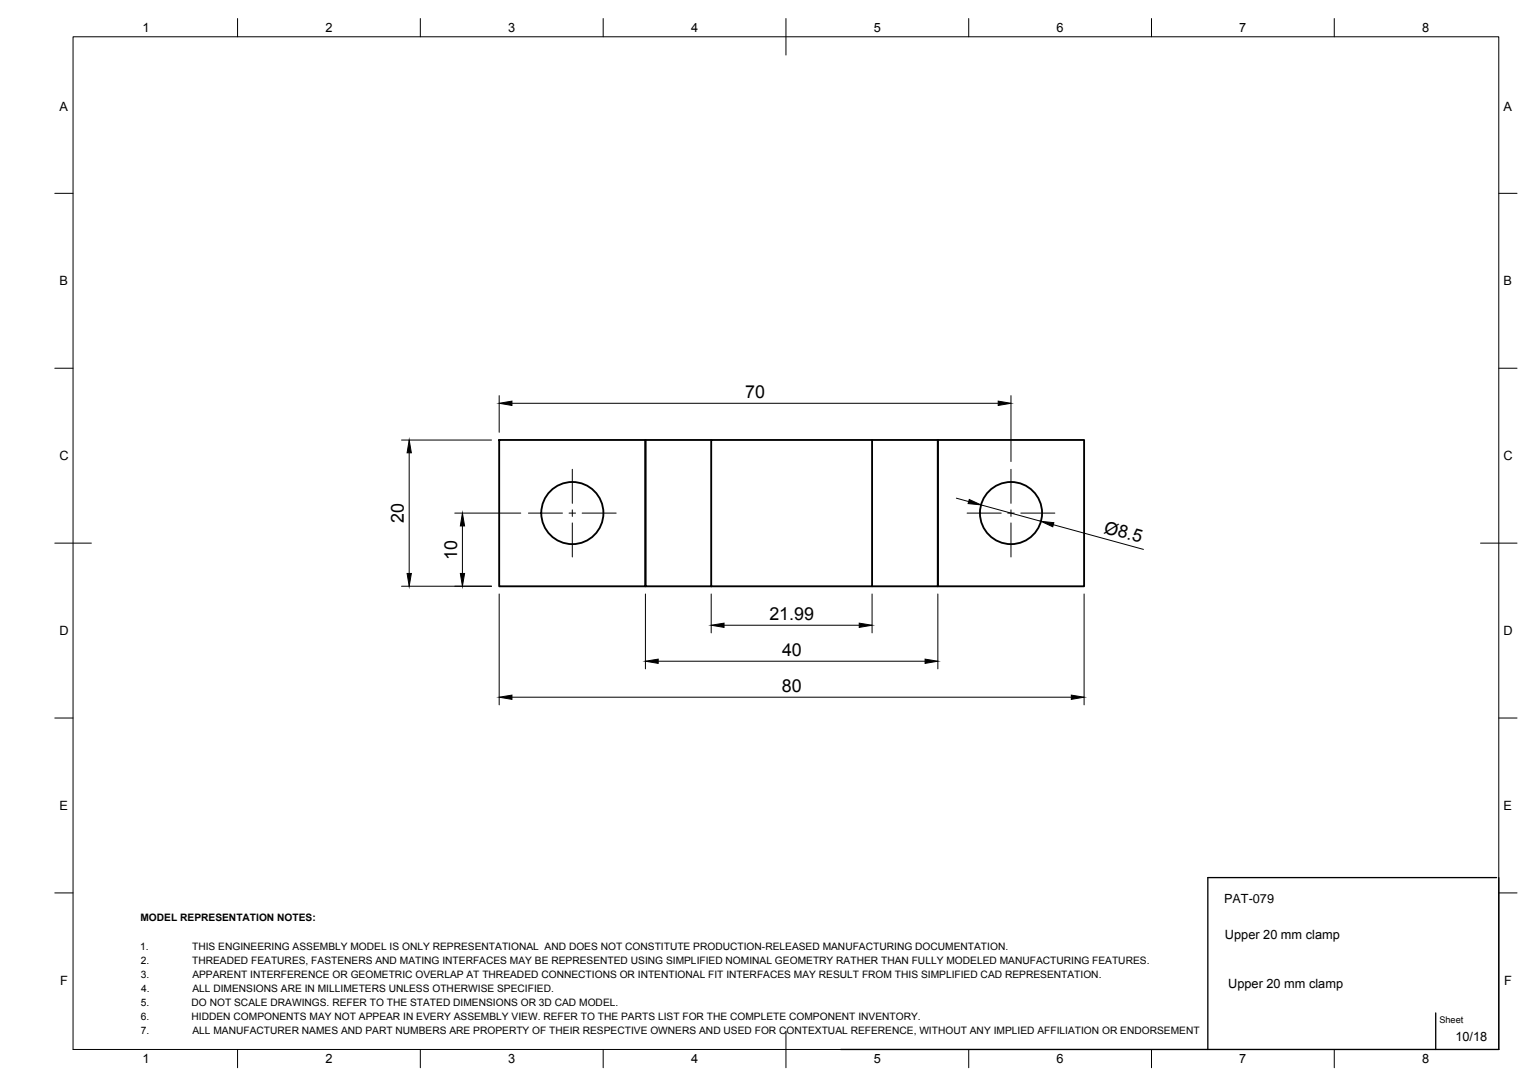
ISO-10303-21;
HEADER;
/* Generated by software containing ST-Developer
 * from STEP Tools, Inc. (www.steptools.com) 
 */

FILE_DESCRIPTION(
/* description */ ('Pipe clamp stand with threaded column'),
/* implementation_level */ '2;1');

FILE_NAME(
/* name */ 'Upper 20 mm clamp.step',
/* time_stamp */ '2026-10-27T10:55:48-07:00',
/* author */ (''),
/* organization */ (''),
/* preprocessor_version */ 'ST-DEVELOPER v20.2',
/* originating_system */ 'Autodesk Translation Framework v15.17.0.0',
/* authorisation */ '');

FILE_SCHEMA (('AUTOMOTIVE_DESIGN { 1 0 10303 214 3 1 1 }'));
ENDSEC;

DATA;
#10=MECHANICAL_DESIGN_GEOMETRIC_PRESENTATION_REPRESENTATION('',(#748,#749,#750),#34433);
#702=SHAPE_REPRESENTATION_RELATIONSHIP('SRR','None',#34544,#724);
#724=ADVANCED_BREP_SHAPE_REPRESENTATION('',(#778,#779,#780),#34412);
#748=STYLED_ITEM('',(#34729),#778);
#749=STYLED_ITEM('',(#34729),#779);
#750=STYLED_ITEM('',(#34729),#780);
#778=MANIFOLD_SOLID_BREP('Body1',#8775);
#779=MANIFOLD_SOLID_BREP('Body2',#8776);
#780=MANIFOLD_SOLID_BREP('Body3',#8777);
#828=FACE_BOUND('',#1821,.T.);
#829=FACE_BOUND('',#1824,.T.);
#830=FACE_BOUND('',#1830,.T.);
#831=FACE_BOUND('',#1833,.T.);
#895=PLANE('',#9352);
#896=PLANE('',#9354);
#897=PLANE('',#9355);
#898=PLANE('',#9358);
#899=PLANE('',#9362);
#900=PLANE('',#9363);
#901=PLANE('',#9364);
#902=PLANE('',#9365);
#903=PLANE('',#9366);
#904=PLANE('',#9367);
#905=PLANE('',#9371);
#906=PLANE('',#9372);
#907=PLANE('',#9373);
#908=PLANE('',#9374);
#909=PLANE('',#9375);
#910=PLANE('',#9376);
#1296=FACE_OUTER_BOUND('',#1812,.T.);
#1297=FACE_OUTER_BOUND('',#1813,.T.);
#1298=FACE_OUTER_BOUND('',#1814,.T.);
#1299=FACE_OUTER_BOUND('',#1815,.T.);
#1300=FACE_OUTER_BOUND('',#1816,.T.);
#1301=FACE_OUTER_BOUND('',#1817,.T.);
#1302=FACE_OUTER_BOUND('',#1818,.T.);
#1303=FACE_OUTER_BOUND('',#1819,.T.);
#1304=FACE_OUTER_BOUND('',#1820,.T.);
#1305=FACE_OUTER_BOUND('',#1822,.T.);
#1306=FACE_OUTER_BOUND('',#1823,.T.);
#1307=FACE_OUTER_BOUND('',#1825,.T.);
#1308=FACE_OUTER_BOUND('',#1826,.T.);
#1309=FACE_OUTER_BOUND('',#1827,.T.);
#1310=FACE_OUTER_BOUND('',#1828,.T.);
#1311=FACE_OUTER_BOUND('',#1829,.T.);
#1312=FACE_OUTER_BOUND('',#1831,.T.);
#1313=FACE_OUTER_BOUND('',#1832,.T.);
#1314=FACE_OUTER_BOUND('',#1834,.T.);
#1315=FACE_OUTER_BOUND('',#1835,.T.);
#1812=EDGE_LOOP('',(#6923,#6924,#6925,#6926));
#1813=EDGE_LOOP('',(#6927,#6928,#6929,#6930));
#1814=EDGE_LOOP('',(#6931,#6932,#6933,#6934));
#1815=EDGE_LOOP('',(#6935,#6936,#6937,#6938));
#1816=EDGE_LOOP('',(#6939,#6940,#6941,#6942));
#1817=EDGE_LOOP('',(#6943,#6944,#6945,#6946));
#1818=EDGE_LOOP('',(#6947,#6948,#6949,#6950));
#1819=EDGE_LOOP('',(#6951,#6952,#6953,#6954));
#1820=EDGE_LOOP('',(#6955,#6956,#6957,#6958));
#1821=EDGE_LOOP('',(#6959));
#1822=EDGE_LOOP('',(#6960,#6961,#6962,#6963));
#1823=EDGE_LOOP('',(#6964,#6965,#6966,#6967));
#1824=EDGE_LOOP('',(#6968));
#1825=EDGE_LOOP('',(#6969,#6970,#6971,#6972));
#1826=EDGE_LOOP('',(#6973,#6974,#6975,#6976));
#1827=EDGE_LOOP('',(#6977,#6978,#6979,#6980));
#1828=EDGE_LOOP('',(#6981,#6982,#6983,#6984));
#1829=EDGE_LOOP('',(#6985,#6986,#6987,#6988));
#1830=EDGE_LOOP('',(#6989));
#1831=EDGE_LOOP('',(#6990,#6991,#6992,#6993));
#1832=EDGE_LOOP('',(#6994,#6995,#6996,#6997));
#1833=EDGE_LOOP('',(#6998));
#1834=EDGE_LOOP('',(#6999,#7000,#7001,#7002));
#1835=EDGE_LOOP('',(#7003,#7004,#7005,#7006));
#2349=LINE('',#28187,#2966);
#2350=LINE('',#28191,#2967);
#2351=LINE('',#28195,#2968);
#2352=LINE('',#28198,#2969);
#2353=LINE('',#28201,#2970);
#2354=LINE('',#28202,#2971);
#2355=LINE('',#28205,#2972);
#2356=LINE('',#28206,#2973);
#2357=LINE('',#28214,#2974);
#2358=LINE('',#28219,#2975);
#2359=LINE('',#28221,#2976);
#2360=LINE('',#28223,#2977);
#2361=LINE('',#28224,#2978);
#2362=LINE('',#28227,#2979);
#2363=LINE('',#28229,#2980);
#2364=LINE('',#28230,#2981);
#2365=LINE('',#28233,#2982);
#2366=LINE('',#28235,#2983);
#2367=LINE('',#28236,#2984);
#2368=LINE('',#28238,#2985);
#2369=LINE('',#28239,#2986);
#2370=LINE('',#28246,#2987);
#2371=LINE('',#28251,#2988);
#2372=LINE('',#28253,#2989);
#2373=LINE('',#28255,#2990);
#2374=LINE('',#28256,#2991);
#2375=LINE('',#28259,#2992);
#2376=LINE('',#28261,#2993);
#2377=LINE('',#28262,#2994);
#2378=LINE('',#28265,#2995);
#2379=LINE('',#28267,#2996);
#2380=LINE('',#28268,#2997);
#2381=LINE('',#28270,#2998);
#2382=LINE('',#28271,#2999);
#2966=VECTOR('',#10612,1.);
#2967=VECTOR('',#10615,1.);
#2968=VECTOR('',#10620,1.);
#2969=VECTOR('',#10623,1.);
#2970=VECTOR('',#10626,1.);
#2971=VECTOR('',#10627,1.);
#2972=VECTOR('',#10630,1.);
#2973=VECTOR('',#10631,1.);
#2974=VECTOR('',#10642,0.425);
#2975=VECTOR('',#10647,1.);
#2976=VECTOR('',#10648,1.);
#2977=VECTOR('',#10649,1.);
#2978=VECTOR('',#10650,1.);
#2979=VECTOR('',#10653,1.);
#2980=VECTOR('',#10654,1.);
#2981=VECTOR('',#10655,1.);
#2982=VECTOR('',#10658,1.);
#2983=VECTOR('',#10659,1.);
#2984=VECTOR('',#10660,1.);
#2985=VECTOR('',#10663,1.);
#2986=VECTOR('',#10664,1.);
#2987=VECTOR('',#10673,0.425);
#2988=VECTOR('',#10678,1.);
#2989=VECTOR('',#10679,1.);
#2990=VECTOR('',#10680,1.);
#2991=VECTOR('',#10681,1.);
#2992=VECTOR('',#10684,1.);
#2993=VECTOR('',#10685,1.);
#2994=VECTOR('',#10686,1.);
#2995=VECTOR('',#10689,1.);
#2996=VECTOR('',#10690,1.);
#2997=VECTOR('',#10691,1.);
#2998=VECTOR('',#10694,1.);
#2999=VECTOR('',#10695,1.);
#3358=CIRCLE('',#9350,1.1);
#3359=CIRCLE('',#9351,1.1);
#3360=CIRCLE('',#9353,2.);
#3361=CIRCLE('',#9357,2.);
#3362=CIRCLE('',#9360,0.425);
#3363=CIRCLE('',#9361,0.425);
#3364=CIRCLE('',#9369,0.425);
#3365=CIRCLE('',#9370,0.425);
#3914=VERTEX_POINT('',#28185);
#3915=VERTEX_POINT('',#28186);
#3916=VERTEX_POINT('',#28188);
#3917=VERTEX_POINT('',#28190);
#3918=VERTEX_POINT('',#28194);
#3919=VERTEX_POINT('',#28196);
#3920=VERTEX_POINT('',#28200);
#3921=VERTEX_POINT('',#28204);
#3922=VERTEX_POINT('',#28211);
#3923=VERTEX_POINT('',#28213);
#3924=VERTEX_POINT('',#28217);
#3925=VERTEX_POINT('',#28218);
#3926=VERTEX_POINT('',#28220);
#3927=VERTEX_POINT('',#28222);
#3928=VERTEX_POINT('',#28226);
#3929=VERTEX_POINT('',#28228);
#3930=VERTEX_POINT('',#28232);
#3931=VERTEX_POINT('',#28234);
#3932=VERTEX_POINT('',#28243);
#3933=VERTEX_POINT('',#28245);
#3934=VERTEX_POINT('',#28249);
#3935=VERTEX_POINT('',#28250);
#3936=VERTEX_POINT('',#28252);
#3937=VERTEX_POINT('',#28254);
#3938=VERTEX_POINT('',#28258);
#3939=VERTEX_POINT('',#28260);
#3940=VERTEX_POINT('',#28264);
#3941=VERTEX_POINT('',#28266);
#4975=EDGE_CURVE('',#3914,#3915,#2349,.T.);
#4976=EDGE_CURVE('',#3916,#3914,#3358,.T.);
#4977=EDGE_CURVE('',#3917,#3916,#2350,.T.);
#4978=EDGE_CURVE('',#3915,#3917,#3359,.T.);
#4979=EDGE_CURVE('',#3914,#3918,#2351,.T.);
#4980=EDGE_CURVE('',#3918,#3919,#3360,.T.);
#4981=EDGE_CURVE('',#3919,#3916,#2352,.T.);
#4982=EDGE_CURVE('',#3920,#3915,#2353,.T.);
#4983=EDGE_CURVE('',#3918,#3920,#2354,.T.);
#4984=EDGE_CURVE('',#3921,#3919,#2355,.T.);
#4985=EDGE_CURVE('',#3917,#3921,#2356,.T.);
#4986=EDGE_CURVE('',#3920,#3921,#3361,.T.);
#4987=EDGE_CURVE('',#3922,#3922,#3362,.T.);
#4988=EDGE_CURVE('',#3922,#3923,#2357,.T.);
#4989=EDGE_CURVE('',#3923,#3923,#3363,.T.);
#4990=EDGE_CURVE('',#3924,#3925,#2358,.T.);
#4991=EDGE_CURVE('',#3924,#3926,#2359,.T.);
#4992=EDGE_CURVE('',#3927,#3926,#2360,.T.);
#4993=EDGE_CURVE('',#3925,#3927,#2361,.T.);
#4994=EDGE_CURVE('',#3925,#3928,#2362,.T.);
#4995=EDGE_CURVE('',#3929,#3927,#2363,.T.);
#4996=EDGE_CURVE('',#3928,#3929,#2364,.T.);
#4997=EDGE_CURVE('',#3928,#3930,#2365,.T.);
#4998=EDGE_CURVE('',#3931,#3929,#2366,.T.);
#4999=EDGE_CURVE('',#3930,#3931,#2367,.T.);
#5000=EDGE_CURVE('',#3930,#3924,#2368,.T.);
#5001=EDGE_CURVE('',#3926,#3931,#2369,.T.);
#5002=EDGE_CURVE('',#3932,#3932,#3364,.T.);
#5003=EDGE_CURVE('',#3932,#3933,#2370,.T.);
#5004=EDGE_CURVE('',#3933,#3933,#3365,.T.);
#5005=EDGE_CURVE('',#3934,#3935,#2371,.T.);
#5006=EDGE_CURVE('',#3934,#3936,#2372,.T.);
#5007=EDGE_CURVE('',#3937,#3936,#2373,.T.);
#5008=EDGE_CURVE('',#3935,#3937,#2374,.T.);
#5009=EDGE_CURVE('',#3935,#3938,#2375,.T.);
#5010=EDGE_CURVE('',#3939,#3937,#2376,.T.);
#5011=EDGE_CURVE('',#3938,#3939,#2377,.T.);
#5012=EDGE_CURVE('',#3938,#3940,#2378,.T.);
#5013=EDGE_CURVE('',#3941,#3939,#2379,.T.);
#5014=EDGE_CURVE('',#3940,#3941,#2380,.T.);
#5015=EDGE_CURVE('',#3940,#3934,#2381,.T.);
#5016=EDGE_CURVE('',#3936,#3941,#2382,.T.);
#6923=ORIENTED_EDGE('',*,*,#4975,.F.);
#6924=ORIENTED_EDGE('',*,*,#4976,.F.);
#6925=ORIENTED_EDGE('',*,*,#4977,.F.);
#6926=ORIENTED_EDGE('',*,*,#4978,.F.);
#6927=ORIENTED_EDGE('',*,*,#4976,.T.);
#6928=ORIENTED_EDGE('',*,*,#4979,.T.);
#6929=ORIENTED_EDGE('',*,*,#4980,.T.);
#6930=ORIENTED_EDGE('',*,*,#4981,.T.);
#6931=ORIENTED_EDGE('',*,*,#4975,.T.);
#6932=ORIENTED_EDGE('',*,*,#4982,.F.);
#6933=ORIENTED_EDGE('',*,*,#4983,.F.);
#6934=ORIENTED_EDGE('',*,*,#4979,.F.);
#6935=ORIENTED_EDGE('',*,*,#4977,.T.);
#6936=ORIENTED_EDGE('',*,*,#4981,.F.);
#6937=ORIENTED_EDGE('',*,*,#4984,.F.);
#6938=ORIENTED_EDGE('',*,*,#4985,.F.);
#6939=ORIENTED_EDGE('',*,*,#4984,.T.);
#6940=ORIENTED_EDGE('',*,*,#4980,.F.);
#6941=ORIENTED_EDGE('',*,*,#4983,.T.);
#6942=ORIENTED_EDGE('',*,*,#4986,.T.);
#6943=ORIENTED_EDGE('',*,*,#4978,.T.);
#6944=ORIENTED_EDGE('',*,*,#4985,.T.);
#6945=ORIENTED_EDGE('',*,*,#4986,.F.);
#6946=ORIENTED_EDGE('',*,*,#4982,.T.);
#6947=ORIENTED_EDGE('',*,*,#4987,.F.);
#6948=ORIENTED_EDGE('',*,*,#4988,.T.);
#6949=ORIENTED_EDGE('',*,*,#4989,.F.);
#6950=ORIENTED_EDGE('',*,*,#4988,.F.);
#6951=ORIENTED_EDGE('',*,*,#4990,.F.);
#6952=ORIENTED_EDGE('',*,*,#4991,.T.);
#6953=ORIENTED_EDGE('',*,*,#4992,.F.);
#6954=ORIENTED_EDGE('',*,*,#4993,.F.);
#6955=ORIENTED_EDGE('',*,*,#4994,.F.);
#6956=ORIENTED_EDGE('',*,*,#4993,.T.);
#6957=ORIENTED_EDGE('',*,*,#4995,.F.);
#6958=ORIENTED_EDGE('',*,*,#4996,.F.);
#6959=ORIENTED_EDGE('',*,*,#4987,.T.);
#6960=ORIENTED_EDGE('',*,*,#4997,.F.);
#6961=ORIENTED_EDGE('',*,*,#4996,.T.);
#6962=ORIENTED_EDGE('',*,*,#4998,.F.);
#6963=ORIENTED_EDGE('',*,*,#4999,.F.);
#6964=ORIENTED_EDGE('',*,*,#5000,.F.);
#6965=ORIENTED_EDGE('',*,*,#4999,.T.);
#6966=ORIENTED_EDGE('',*,*,#5001,.F.);
#6967=ORIENTED_EDGE('',*,*,#4991,.F.);
#6968=ORIENTED_EDGE('',*,*,#4989,.T.);
#6969=ORIENTED_EDGE('',*,*,#5001,.T.);
#6970=ORIENTED_EDGE('',*,*,#4998,.T.);
#6971=ORIENTED_EDGE('',*,*,#4995,.T.);
#6972=ORIENTED_EDGE('',*,*,#4992,.T.);
#6973=ORIENTED_EDGE('',*,*,#5000,.T.);
#6974=ORIENTED_EDGE('',*,*,#4990,.T.);
#6975=ORIENTED_EDGE('',*,*,#4994,.T.);
#6976=ORIENTED_EDGE('',*,*,#4997,.T.);
#6977=ORIENTED_EDGE('',*,*,#5002,.F.);
#6978=ORIENTED_EDGE('',*,*,#5003,.T.);
#6979=ORIENTED_EDGE('',*,*,#5004,.F.);
#6980=ORIENTED_EDGE('',*,*,#5003,.F.);
#6981=ORIENTED_EDGE('',*,*,#5005,.F.);
#6982=ORIENTED_EDGE('',*,*,#5006,.T.);
#6983=ORIENTED_EDGE('',*,*,#5007,.F.);
#6984=ORIENTED_EDGE('',*,*,#5008,.F.);
#6985=ORIENTED_EDGE('',*,*,#5009,.F.);
#6986=ORIENTED_EDGE('',*,*,#5008,.T.);
#6987=ORIENTED_EDGE('',*,*,#5010,.F.);
#6988=ORIENTED_EDGE('',*,*,#5011,.F.);
#6989=ORIENTED_EDGE('',*,*,#5002,.T.);
#6990=ORIENTED_EDGE('',*,*,#5012,.F.);
#6991=ORIENTED_EDGE('',*,*,#5011,.T.);
#6992=ORIENTED_EDGE('',*,*,#5013,.F.);
#6993=ORIENTED_EDGE('',*,*,#5014,.F.);
#6994=ORIENTED_EDGE('',*,*,#5015,.F.);
#6995=ORIENTED_EDGE('',*,*,#5014,.T.);
#6996=ORIENTED_EDGE('',*,*,#5016,.F.);
#6997=ORIENTED_EDGE('',*,*,#5006,.F.);
#6998=ORIENTED_EDGE('',*,*,#5004,.T.);
#6999=ORIENTED_EDGE('',*,*,#5016,.T.);
#7000=ORIENTED_EDGE('',*,*,#5013,.T.);
#7001=ORIENTED_EDGE('',*,*,#5010,.T.);
#7002=ORIENTED_EDGE('',*,*,#5007,.T.);
#7003=ORIENTED_EDGE('',*,*,#5015,.T.);
#7004=ORIENTED_EDGE('',*,*,#5005,.T.);
#7005=ORIENTED_EDGE('',*,*,#5009,.T.);
#7006=ORIENTED_EDGE('',*,*,#5012,.T.);
#8211=CYLINDRICAL_SURFACE('',#9349,1.1);
#8212=CYLINDRICAL_SURFACE('',#9356,2.);
#8213=CYLINDRICAL_SURFACE('',#9359,0.425);
#8214=CYLINDRICAL_SURFACE('',#9368,0.425);
#8533=ADVANCED_FACE('',(#1296),#8211,.F.);
#8534=ADVANCED_FACE('',(#1297),#895,.T.);
#8535=ADVANCED_FACE('',(#1298),#896,.F.);
#8536=ADVANCED_FACE('',(#1299),#897,.F.);
#8537=ADVANCED_FACE('',(#1300),#8212,.T.);
#8538=ADVANCED_FACE('',(#1301),#898,.F.);
#8539=ADVANCED_FACE('',(#1302),#8213,.F.);
#8540=ADVANCED_FACE('',(#1303),#899,.T.);
#8541=ADVANCED_FACE('',(#1304,#828),#900,.T.);
#8542=ADVANCED_FACE('',(#1305),#901,.T.);
#8543=ADVANCED_FACE('',(#1306,#829),#902,.T.);
#8544=ADVANCED_FACE('',(#1307),#903,.T.);
#8545=ADVANCED_FACE('',(#1308),#904,.F.);
#8546=ADVANCED_FACE('',(#1309),#8214,.F.);
#8547=ADVANCED_FACE('',(#1310),#905,.T.);
#8548=ADVANCED_FACE('',(#1311,#830),#906,.T.);
#8549=ADVANCED_FACE('',(#1312),#907,.T.);
#8550=ADVANCED_FACE('',(#1313,#831),#908,.T.);
#8551=ADVANCED_FACE('',(#1314),#909,.T.);
#8552=ADVANCED_FACE('',(#1315),#910,.F.);
#8775=CLOSED_SHELL('',(#8533,#8534,#8535,#8536,#8537,#8538));
#8776=CLOSED_SHELL('',(#8539,#8540,#8541,#8542,#8543,#8544,#8545));
#8777=CLOSED_SHELL('',(#8546,#8547,#8548,#8549,#8550,#8551,#8552));
#9348=AXIS2_PLACEMENT_3D('',#28183,#10608,#10609);
#9349=AXIS2_PLACEMENT_3D('',#28184,#10610,#10611);
#9350=AXIS2_PLACEMENT_3D('',#28189,#10613,#10614);
#9351=AXIS2_PLACEMENT_3D('',#28192,#10616,#10617);
#9352=AXIS2_PLACEMENT_3D('',#28193,#10618,#10619);
#9353=AXIS2_PLACEMENT_3D('',#28197,#10621,#10622);
#9354=AXIS2_PLACEMENT_3D('',#28199,#10624,#10625);
#9355=AXIS2_PLACEMENT_3D('',#28203,#10628,#10629);
#9356=AXIS2_PLACEMENT_3D('',#28207,#10632,#10633);
#9357=AXIS2_PLACEMENT_3D('',#28208,#10634,#10635);
#9358=AXIS2_PLACEMENT_3D('',#28209,#10636,#10637);
#9359=AXIS2_PLACEMENT_3D('',#28210,#10638,#10639);
#9360=AXIS2_PLACEMENT_3D('',#28212,#10640,#10641);
#9361=AXIS2_PLACEMENT_3D('',#28215,#10643,#10644);
#9362=AXIS2_PLACEMENT_3D('',#28216,#10645,#10646);
#9363=AXIS2_PLACEMENT_3D('',#28225,#10651,#10652);
#9364=AXIS2_PLACEMENT_3D('',#28231,#10656,#10657);
#9365=AXIS2_PLACEMENT_3D('',#28237,#10661,#10662);
#9366=AXIS2_PLACEMENT_3D('',#28240,#10665,#10666);
#9367=AXIS2_PLACEMENT_3D('',#28241,#10667,#10668);
#9368=AXIS2_PLACEMENT_3D('',#28242,#10669,#10670);
#9369=AXIS2_PLACEMENT_3D('',#28244,#10671,#10672);
#9370=AXIS2_PLACEMENT_3D('',#28247,#10674,#10675);
#9371=AXIS2_PLACEMENT_3D('',#28248,#10676,#10677);
#9372=AXIS2_PLACEMENT_3D('',#28257,#10682,#10683);
#9373=AXIS2_PLACEMENT_3D('',#28263,#10687,#10688);
#9374=AXIS2_PLACEMENT_3D('',#28269,#10692,#10693);
#9375=AXIS2_PLACEMENT_3D('',#28272,#10696,#10697);
#9376=AXIS2_PLACEMENT_3D('',#28273,#10698,#10699);
#10608=DIRECTION('axis',(0.,0.,1.));
#10609=DIRECTION('refdir',(1.,0.,0.));
#10610=DIRECTION('center_axis',(0.,1.,0.));
#10611=DIRECTION('ref_axis',(1.,0.,0.));
#10612=DIRECTION('',(0.,-1.,0.));
#10613=DIRECTION('center_axis',(0.,-1.,0.));
#10614=DIRECTION('ref_axis',(1.,0.,0.));
#10615=DIRECTION('',(0.,1.,0.));
#10616=DIRECTION('center_axis',(0.,1.,0.));
#10617=DIRECTION('ref_axis',(1.,0.,0.));
#10618=DIRECTION('center_axis',(0.,1.,0.));
#10619=DIRECTION('ref_axis',(1.,0.,0.));
#10620=DIRECTION('',(-1.,0.,0.));
#10621=DIRECTION('center_axis',(0.,1.,0.));
#10622=DIRECTION('ref_axis',(1.,0.,0.));
#10623=DIRECTION('',(-1.,0.,0.));
#10624=DIRECTION('center_axis',(0.,0.,1.));
#10625=DIRECTION('ref_axis',(1.,0.,0.));
#10626=DIRECTION('',(1.,0.,0.));
#10627=DIRECTION('',(0.,-1.,0.));
#10628=DIRECTION('center_axis',(0.,0.,1.));
#10629=DIRECTION('ref_axis',(1.,0.,0.));
#10630=DIRECTION('',(0.,1.,0.));
#10631=DIRECTION('',(1.,0.,0.));
#10632=DIRECTION('center_axis',(0.,1.,0.));
#10633=DIRECTION('ref_axis',(1.,0.,0.));
#10634=DIRECTION('center_axis',(0.,1.,0.));
#10635=DIRECTION('ref_axis',(1.,0.,0.));
#10636=DIRECTION('center_axis',(0.,1.,0.));
#10637=DIRECTION('ref_axis',(1.,0.,0.));
#10638=DIRECTION('center_axis',(0.,0.,1.));
#10639=DIRECTION('ref_axis',(1.,0.,0.));
#10640=DIRECTION('center_axis',(0.,0.,1.));
#10641=DIRECTION('ref_axis',(1.,0.,0.));
#10642=DIRECTION('',(0.,0.,1.));
#10643=DIRECTION('center_axis',(0.,0.,-1.));
#10644=DIRECTION('ref_axis',(1.,0.,0.));
#10645=DIRECTION('center_axis',(-1.,0.,0.));
#10646=DIRECTION('ref_axis',(0.,0.,1.));
#10647=DIRECTION('',(0.,0.,-1.));
#10648=DIRECTION('',(0.,1.,0.));
#10649=DIRECTION('',(0.,0.,1.));
#10650=DIRECTION('',(0.,1.,0.));
#10651=DIRECTION('center_axis',(0.,0.,-1.));
#10652=DIRECTION('ref_axis',(-1.,0.,0.));
#10653=DIRECTION('',(1.,0.,0.));
#10654=DIRECTION('',(-1.,0.,0.));
#10655=DIRECTION('',(0.,1.,0.));
#10656=DIRECTION('center_axis',(1.,0.,0.));
#10657=DIRECTION('ref_axis',(0.,0.,-1.));
#10658=DIRECTION('',(0.,0.,1.));
#10659=DIRECTION('',(0.,0.,-1.));
#10660=DIRECTION('',(0.,1.,0.));
#10661=DIRECTION('center_axis',(0.,0.,1.));
#10662=DIRECTION('ref_axis',(1.,0.,0.));
#10663=DIRECTION('',(-1.,0.,0.));
#10664=DIRECTION('',(1.,0.,0.));
#10665=DIRECTION('center_axis',(0.,1.,0.));
#10666=DIRECTION('ref_axis',(0.,0.,1.));
#10667=DIRECTION('center_axis',(0.,1.,0.));
#10668=DIRECTION('ref_axis',(1.,0.,0.));
#10669=DIRECTION('center_axis',(0.,0.,1.));
#10670=DIRECTION('ref_axis',(1.,0.,0.));
#10671=DIRECTION('center_axis',(0.,0.,1.));
#10672=DIRECTION('ref_axis',(1.,0.,0.));
#10673=DIRECTION('',(0.,0.,1.));
#10674=DIRECTION('center_axis',(0.,0.,-1.));
#10675=DIRECTION('ref_axis',(1.,0.,0.));
#10676=DIRECTION('center_axis',(-1.,0.,0.));
#10677=DIRECTION('ref_axis',(0.,0.,1.));
#10678=DIRECTION('',(0.,0.,-1.));
#10679=DIRECTION('',(0.,1.,0.));
#10680=DIRECTION('',(0.,0.,1.));
#10681=DIRECTION('',(0.,1.,0.));
#10682=DIRECTION('center_axis',(0.,0.,-1.));
#10683=DIRECTION('ref_axis',(-1.,0.,0.));
#10684=DIRECTION('',(1.,0.,0.));
#10685=DIRECTION('',(-1.,0.,0.));
#10686=DIRECTION('',(0.,1.,0.));
#10687=DIRECTION('center_axis',(1.,0.,0.));
#10688=DIRECTION('ref_axis',(0.,0.,-1.));
#10689=DIRECTION('',(0.,0.,1.));
#10690=DIRECTION('',(0.,0.,-1.));
#10691=DIRECTION('',(0.,1.,0.));
#10692=DIRECTION('center_axis',(0.,0.,1.));
#10693=DIRECTION('ref_axis',(1.,0.,0.));
#10694=DIRECTION('',(-1.,0.,0.));
#10695=DIRECTION('',(1.,0.,0.));
#10696=DIRECTION('center_axis',(0.,1.,0.));
#10697=DIRECTION('ref_axis',(0.,0.,1.));
#10698=DIRECTION('center_axis',(0.,1.,0.));
#10699=DIRECTION('ref_axis',(1.,0.,0.));
#28183=CARTESIAN_POINT('',(0.,0.,0.));
#28184=CARTESIAN_POINT('Origin',(0.,-1.1,18.));
#28185=CARTESIAN_POINT('',(-1.09971587239614,1.,18.025));
#28186=CARTESIAN_POINT('',(-1.09971587239614,-1.,18.025));
#28187=CARTESIAN_POINT('',(-1.09971587239614,-1.1,18.025));
#28188=CARTESIAN_POINT('',(1.09971587239614,1.,18.025));
#28189=CARTESIAN_POINT('Origin',(0.,1.,18.));
#28190=CARTESIAN_POINT('',(1.09971587239614,-1.,18.025));
#28191=CARTESIAN_POINT('',(1.09971587239614,-1.1,18.025));
#28192=CARTESIAN_POINT('Origin',(0.,-1.,18.));
#28193=CARTESIAN_POINT('Origin',(0.,1.,18.));
#28194=CARTESIAN_POINT('',(-1.99984374389601,1.,18.025));
#28195=CARTESIAN_POINT('',(-2.,1.,18.025));
#28196=CARTESIAN_POINT('',(1.99984374389601,1.,18.025));
#28197=CARTESIAN_POINT('Origin',(0.,1.,18.));
#28198=CARTESIAN_POINT('',(-2.,1.,18.025));
#28199=CARTESIAN_POINT('Origin',(-4.,-1.1,18.025));
#28200=CARTESIAN_POINT('',(-1.99984374389601,-1.,18.025));
#28201=CARTESIAN_POINT('',(-2.,-1.,18.025));
#28202=CARTESIAN_POINT('',(-1.99984374389601,-1.,18.025));
#28203=CARTESIAN_POINT('Origin',(-4.,-1.1,18.025));
#28204=CARTESIAN_POINT('',(1.99984374389601,-1.,18.025));
#28205=CARTESIAN_POINT('',(1.99984374389601,-1.,18.025));
#28206=CARTESIAN_POINT('',(-2.,-1.,18.025));
#28207=CARTESIAN_POINT('Origin',(0.,-1.,18.));
#28208=CARTESIAN_POINT('Origin',(0.,-1.,18.));
#28209=CARTESIAN_POINT('Origin',(0.,-1.,18.));
#28210=CARTESIAN_POINT('Origin',(-3.,0.,16.7));
#28211=CARTESIAN_POINT('',(-3.425,-5.20474889637625E-17,18.025));
#28212=CARTESIAN_POINT('Origin',(-3.,0.,18.025));
#28213=CARTESIAN_POINT('',(-3.425,5.20474889637625E-17,19.2));
#28214=CARTESIAN_POINT('',(-3.425,-5.20474889637625E-17,16.7));
#28215=CARTESIAN_POINT('Origin',(-3.,0.,19.2));
#28216=CARTESIAN_POINT('Origin',(-4.,-1.,18.025));
#28217=CARTESIAN_POINT('',(-4.,-1.,19.2));
#28218=CARTESIAN_POINT('',(-4.,-1.,18.025));
#28219=CARTESIAN_POINT('',(-4.,-1.,19.2));
#28220=CARTESIAN_POINT('',(-4.,1.,19.2));
#28221=CARTESIAN_POINT('',(-4.,-1.,19.2));
#28222=CARTESIAN_POINT('',(-4.,1.,18.025));
#28223=CARTESIAN_POINT('',(-4.,1.,19.2));
#28224=CARTESIAN_POINT('',(-4.,-1.,18.025));
#28225=CARTESIAN_POINT('Origin',(-2.,-1.,18.025));
#28226=CARTESIAN_POINT('',(-2.,-1.,18.025));
#28227=CARTESIAN_POINT('',(-4.,-1.,18.025));
#28228=CARTESIAN_POINT('',(-2.,1.,18.025));
#28229=CARTESIAN_POINT('',(-4.,1.,18.025));
#28230=CARTESIAN_POINT('',(-2.,-1.,18.025));
#28231=CARTESIAN_POINT('Origin',(-2.,-1.,19.2));
#28232=CARTESIAN_POINT('',(-2.,-1.,19.2));
#28233=CARTESIAN_POINT('',(-2.,-1.,18.025));
#28234=CARTESIAN_POINT('',(-2.,1.,19.2));
#28235=CARTESIAN_POINT('',(-2.,1.,18.025));
#28236=CARTESIAN_POINT('',(-2.,-1.,19.2));
#28237=CARTESIAN_POINT('Origin',(-4.,-1.,19.2));
#28238=CARTESIAN_POINT('',(-2.,-1.,19.2));
#28239=CARTESIAN_POINT('',(-2.,1.,19.2));
#28240=CARTESIAN_POINT('Origin',(-3.,1.,18.6125));
#28241=CARTESIAN_POINT('Origin',(-3.,-1.,18.6125));
#28242=CARTESIAN_POINT('Origin',(3.,0.,16.7));
#28243=CARTESIAN_POINT('',(2.575,-5.20474889637625E-17,18.025));
#28244=CARTESIAN_POINT('Origin',(3.,0.,18.025));
#28245=CARTESIAN_POINT('',(2.575,5.20474889637625E-17,19.2));
#28246=CARTESIAN_POINT('',(2.575,-5.20474889637625E-17,16.7));
#28247=CARTESIAN_POINT('Origin',(3.,0.,19.2));
#28248=CARTESIAN_POINT('Origin',(2.,-1.,18.025));
#28249=CARTESIAN_POINT('',(2.,-1.,19.2));
#28250=CARTESIAN_POINT('',(2.,-1.,18.025));
#28251=CARTESIAN_POINT('',(2.,-1.,19.2));
#28252=CARTESIAN_POINT('',(2.,1.,19.2));
#28253=CARTESIAN_POINT('',(2.,-1.,19.2));
#28254=CARTESIAN_POINT('',(2.,1.,18.025));
#28255=CARTESIAN_POINT('',(2.,1.,19.2));
#28256=CARTESIAN_POINT('',(2.,-1.,18.025));
#28257=CARTESIAN_POINT('Origin',(4.,-1.,18.025));
#28258=CARTESIAN_POINT('',(4.,-1.,18.025));
#28259=CARTESIAN_POINT('',(2.,-1.,18.025));
#28260=CARTESIAN_POINT('',(4.,1.,18.025));
#28261=CARTESIAN_POINT('',(2.,1.,18.025));
#28262=CARTESIAN_POINT('',(4.,-1.,18.025));
#28263=CARTESIAN_POINT('Origin',(4.,-1.,19.2));
#28264=CARTESIAN_POINT('',(4.,-1.,19.2));
#28265=CARTESIAN_POINT('',(4.,-1.,18.025));
#28266=CARTESIAN_POINT('',(4.,1.,19.2));
#28267=CARTESIAN_POINT('',(4.,1.,18.025));
#28268=CARTESIAN_POINT('',(4.,-1.,19.2));
#28269=CARTESIAN_POINT('Origin',(2.,-1.,19.2));
#28270=CARTESIAN_POINT('',(4.,-1.,19.2));
#28271=CARTESIAN_POINT('',(4.,1.,19.2));
#28272=CARTESIAN_POINT('Origin',(3.,1.,18.6125));
#28273=CARTESIAN_POINT('Origin',(3.,-1.,18.6125));
#34383=UNCERTAINTY_MEASURE_WITH_UNIT(LENGTH_MEASURE(0.001),#34434,
'DISTANCE_ACCURACY_VALUE',
'Maximum model space distance between geometric entities at asserted c
onnectivities');
#34404=UNCERTAINTY_MEASURE_WITH_UNIT(LENGTH_MEASURE(0.001),#34434,
'DISTANCE_ACCURACY_VALUE',
'Maximum model space distance between geometric entities at asserted c
onnectivities');
#34412=(
GEOMETRIC_REPRESENTATION_CONTEXT(3)
GLOBAL_UNCERTAINTY_ASSIGNED_CONTEXT((#34383))
GLOBAL_UNIT_ASSIGNED_CONTEXT((#34434,#34436,#34437))
REPRESENTATION_CONTEXT('','3D')
);
#34433=(
GEOMETRIC_REPRESENTATION_CONTEXT(3)
GLOBAL_UNCERTAINTY_ASSIGNED_CONTEXT((#34404))
GLOBAL_UNIT_ASSIGNED_CONTEXT((#34434,#34436,#34437))
REPRESENTATION_CONTEXT('','3D')
);
#34434=(
LENGTH_UNIT()
NAMED_UNIT(*)
SI_UNIT(.CENTI.,.METRE.)
);
#34436=(
NAMED_UNIT(*)
PLANE_ANGLE_UNIT()
SI_UNIT($,.RADIAN.)
);
#34437=(
NAMED_UNIT(*)
SI_UNIT($,.STERADIAN.)
SOLID_ANGLE_UNIT()
);
#34445=SHAPE_DEFINITION_REPRESENTATION(#34473,#34544);
#34473=PRODUCT_DEFINITION_SHAPE('',$,#34573);
#34544=SHAPE_REPRESENTATION('',(#9348),#34412);
#34565=PRODUCT_DEFINITION_CONTEXT('part definition',#34651,'design');
#34573=PRODUCT_DEFINITION('Upper 20 mm clamp','Upper 20 mm clamp',#34601,
#34565);
#34601=PRODUCT_DEFINITION_FORMATION('',$,#34660);
#34651=APPLICATION_CONTEXT(
'Core Data for Automotive Mechanical Design Process');
#34652=PRODUCT_CONTEXT('part definition',#34651,'mechanical');
#34660=PRODUCT('Upper 20 mm clamp','Upper 20 mm clamp',
'Upper 20 mm clamp',(#34652));
#34723=COLOUR_RGB('Light Blue',0.38,0.62,0.78);
#34724=FILL_AREA_STYLE_COLOUR('',#34723);
#34725=FILL_AREA_STYLE('',(#34724));
#34726=SURFACE_STYLE_FILL_AREA(#34725);
#34727=SURFACE_SIDE_STYLE('',(#34726));
#34728=SURFACE_STYLE_USAGE(.BOTH.,#34727);
#34729=PRESENTATION_STYLE_ASSIGNMENT((#34728));
ENDSEC;
END-ISO-10303-21;
